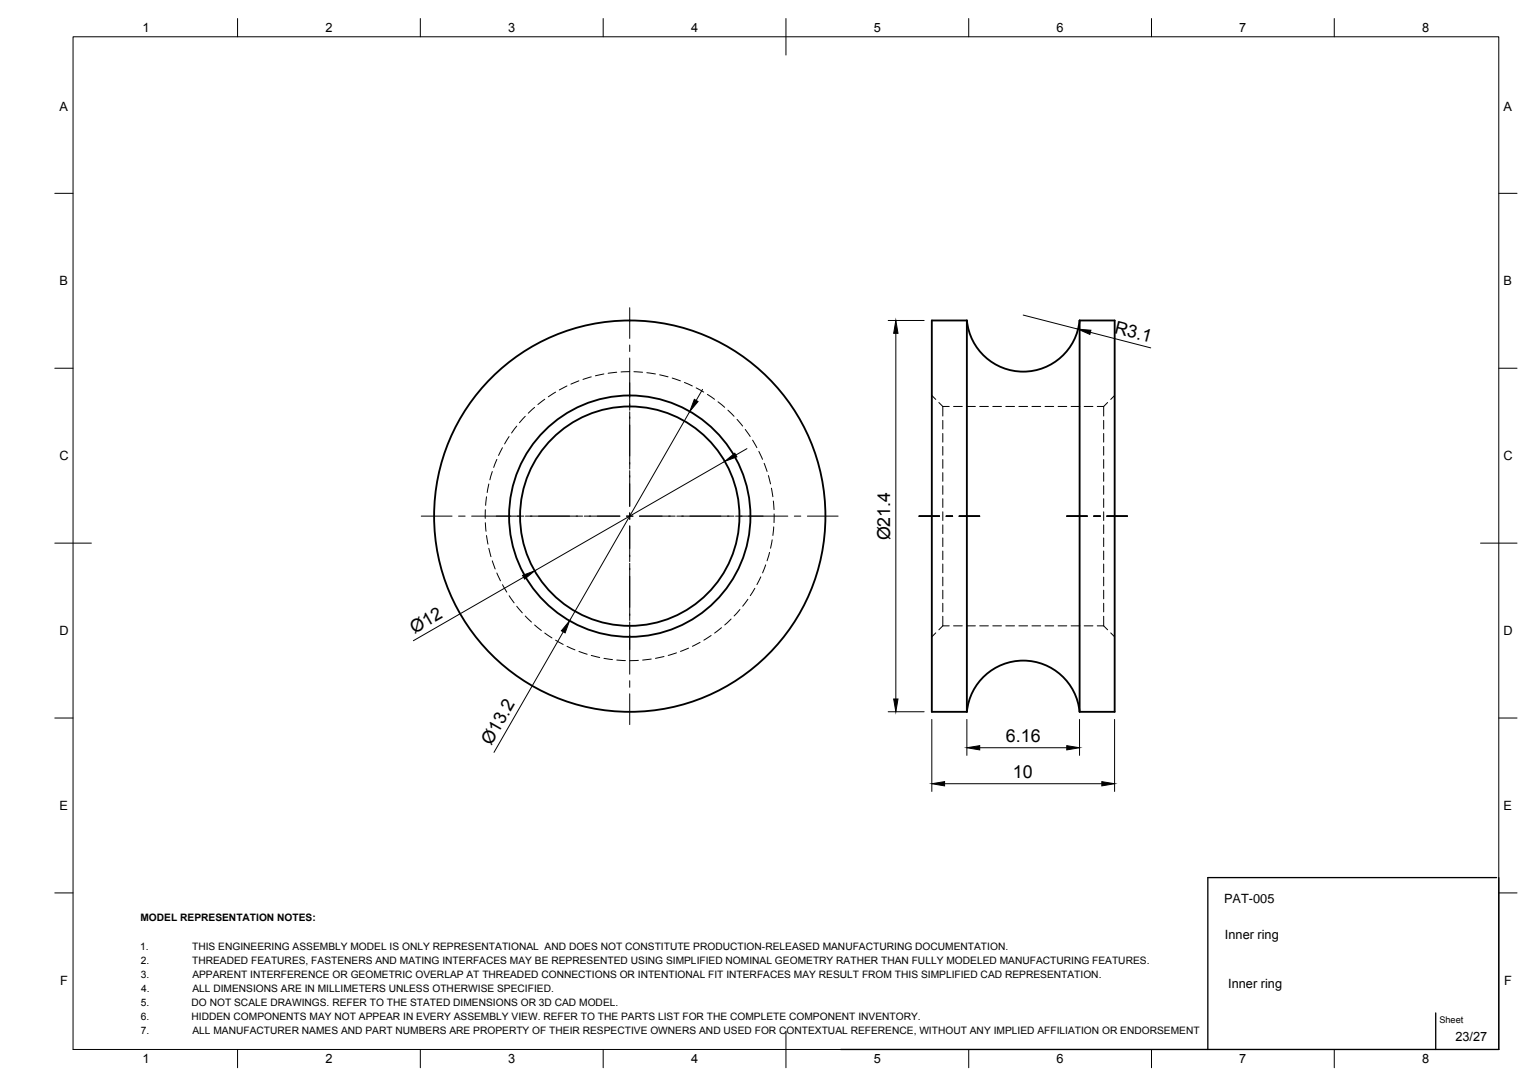
ISO-10303-21;
HEADER;
/* Generated by software containing ST-Developer
 * from STEP Tools, Inc. (www.steptools.com) 
 */

FILE_DESCRIPTION(
/* description */ ('Ball-race swivel caster'),
/* implementation_level */ '2;1');

FILE_NAME(
/* name */ 'Inner ring.step',
/* time_stamp */ '2026-10-29T16:15:51-07:00',
/* author */ (''),
/* organization */ (''),
/* preprocessor_version */ 'ST-DEVELOPER v20.2',
/* originating_system */ 'Autodesk Translation Framework v15.17.0.0',
/* authorisation */ '');

FILE_SCHEMA (('AUTOMOTIVE_DESIGN { 1 0 10303 214 3 1 1 }'));
ENDSEC;

DATA;
#10=MECHANICAL_DESIGN_GEOMETRIC_PRESENTATION_REPRESENTATION('',(#321),#7816);
#30=CONICAL_SURFACE('',#4357,0.63,0.785398163397448);
#31=CONICAL_SURFACE('',#4364,0.63,0.785398163397448);
#190=TOROIDAL_SURFACE('',#4346,1.1,0.309556);
#272=SHAPE_REPRESENTATION_RELATIONSHIP('SRR','None',#7921,#292);
#292=ADVANCED_BREP_SHAPE_REPRESENTATION('',(#356),#7810);
#321=STYLED_ITEM('',(#8097),#356);
#356=MANIFOLD_SOLID_BREP('Body1',#3728);
#427=FACE_BOUND('',#953,.T.);
#428=FACE_BOUND('',#956,.T.);
#506=PLANE('',#4359);
#507=PLANE('',#4362);
#681=FACE_OUTER_BOUND('',#948,.T.);
#682=FACE_OUTER_BOUND('',#949,.T.);
#683=FACE_OUTER_BOUND('',#950,.T.);
#684=FACE_OUTER_BOUND('',#951,.T.);
#685=FACE_OUTER_BOUND('',#952,.T.);
#686=FACE_OUTER_BOUND('',#954,.T.);
#687=FACE_OUTER_BOUND('',#955,.T.);
#688=FACE_OUTER_BOUND('',#957,.T.);
#948=EDGE_LOOP('',(#3217,#3218,#3219,#3220,#3221,#3222));
#949=EDGE_LOOP('',(#3223,#3224,#3225,#3226,#3227));
#950=EDGE_LOOP('',(#3228,#3229,#3230,#3231));
#951=EDGE_LOOP('',(#3232,#3233,#3234,#3235));
#952=EDGE_LOOP('',(#3236));
#953=EDGE_LOOP('',(#3237));
#954=EDGE_LOOP('',(#3238,#3239,#3240,#3241,#3242));
#955=EDGE_LOOP('',(#3243));
#956=EDGE_LOOP('',(#3244));
#957=EDGE_LOOP('',(#3245,#3246,#3247,#3248));
#1148=LINE('',#7228,#1303);
#1149=LINE('',#7234,#1304);
#1150=LINE('',#7238,#1305);
#1151=LINE('',#7244,#1306);
#1152=LINE('',#7249,#1307);
#1303=VECTOR('',#5408,1.070235);
#1304=VECTOR('',#5415,0.6);
#1305=VECTOR('',#5420,0.63);
#1306=VECTOR('',#5429,1.070235);
#1307=VECTOR('',#5436,0.63);
#1512=CIRCLE('',#4347,1.070235);
#1513=CIRCLE('',#4348,1.070235);
#1514=CIRCLE('',#4349,0.309556);
#1515=CIRCLE('',#4350,1.070235);
#1516=CIRCLE('',#4351,1.070235);
#1517=CIRCLE('',#4353,1.070235);
#1518=CIRCLE('',#4355,0.6);
#1519=CIRCLE('',#4356,0.6);
#1520=CIRCLE('',#4358,0.66);
#1521=CIRCLE('',#4361,1.070235);
#1522=CIRCLE('',#4363,0.66);
#1858=VERTEX_POINT('',#7217);
#1859=VERTEX_POINT('',#7218);
#1860=VERTEX_POINT('',#7221);
#1861=VERTEX_POINT('',#7223);
#1862=VERTEX_POINT('',#7227);
#1863=VERTEX_POINT('',#7231);
#1864=VERTEX_POINT('',#7233);
#1865=VERTEX_POINT('',#7237);
#1866=VERTEX_POINT('',#7242);
#1867=VERTEX_POINT('',#7246);
#2328=EDGE_CURVE('',#1858,#1859,#1512,.T.);
#2329=EDGE_CURVE('',#1859,#1858,#1513,.T.);
#2330=EDGE_CURVE('',#1859,#1860,#1514,.T.);
#2331=EDGE_CURVE('',#1861,#1860,#1515,.T.);
#2332=EDGE_CURVE('',#1860,#1861,#1516,.T.);
#2333=EDGE_CURVE('',#1861,#1862,#1148,.T.);
#2334=EDGE_CURVE('',#1862,#1862,#1517,.T.);
#2335=EDGE_CURVE('',#1863,#1863,#1518,.T.);
#2336=EDGE_CURVE('',#1863,#1864,#1149,.T.);
#2337=EDGE_CURVE('',#1864,#1864,#1519,.T.);
#2338=EDGE_CURVE('',#1864,#1865,#1150,.T.);
#2339=EDGE_CURVE('',#1865,#1865,#1520,.T.);
#2340=EDGE_CURVE('',#1866,#1866,#1521,.T.);
#2341=EDGE_CURVE('',#1866,#1858,#1151,.T.);
#2342=EDGE_CURVE('',#1867,#1867,#1522,.T.);
#2343=EDGE_CURVE('',#1867,#1863,#1152,.T.);
#3217=ORIENTED_EDGE('',*,*,#2328,.F.);
#3218=ORIENTED_EDGE('',*,*,#2329,.F.);
#3219=ORIENTED_EDGE('',*,*,#2330,.T.);
#3220=ORIENTED_EDGE('',*,*,#2331,.F.);
#3221=ORIENTED_EDGE('',*,*,#2332,.F.);
#3222=ORIENTED_EDGE('',*,*,#2330,.F.);
#3223=ORIENTED_EDGE('',*,*,#2331,.T.);
#3224=ORIENTED_EDGE('',*,*,#2332,.T.);
#3225=ORIENTED_EDGE('',*,*,#2333,.T.);
#3226=ORIENTED_EDGE('',*,*,#2334,.T.);
#3227=ORIENTED_EDGE('',*,*,#2333,.F.);
#3228=ORIENTED_EDGE('',*,*,#2335,.T.);
#3229=ORIENTED_EDGE('',*,*,#2336,.T.);
#3230=ORIENTED_EDGE('',*,*,#2337,.F.);
#3231=ORIENTED_EDGE('',*,*,#2336,.F.);
#3232=ORIENTED_EDGE('',*,*,#2337,.T.);
#3233=ORIENTED_EDGE('',*,*,#2338,.T.);
#3234=ORIENTED_EDGE('',*,*,#2339,.F.);
#3235=ORIENTED_EDGE('',*,*,#2338,.F.);
#3236=ORIENTED_EDGE('',*,*,#2334,.F.);
#3237=ORIENTED_EDGE('',*,*,#2339,.T.);
#3238=ORIENTED_EDGE('',*,*,#2340,.F.);
#3239=ORIENTED_EDGE('',*,*,#2341,.T.);
#3240=ORIENTED_EDGE('',*,*,#2328,.T.);
#3241=ORIENTED_EDGE('',*,*,#2329,.T.);
#3242=ORIENTED_EDGE('',*,*,#2341,.F.);
#3243=ORIENTED_EDGE('',*,*,#2340,.T.);
#3244=ORIENTED_EDGE('',*,*,#2342,.F.);
#3245=ORIENTED_EDGE('',*,*,#2342,.T.);
#3246=ORIENTED_EDGE('',*,*,#2343,.T.);
#3247=ORIENTED_EDGE('',*,*,#2335,.F.);
#3248=ORIENTED_EDGE('',*,*,#2343,.F.);
#3481=CYLINDRICAL_SURFACE('',#4352,1.070235);
#3482=CYLINDRICAL_SURFACE('',#4354,0.6);
#3483=CYLINDRICAL_SURFACE('',#4360,1.070235);
#3652=ADVANCED_FACE('',(#681),#190,.F.);
#3653=ADVANCED_FACE('',(#682),#3481,.T.);
#3654=ADVANCED_FACE('',(#683),#3482,.F.);
#3655=ADVANCED_FACE('',(#684),#30,.F.);
#3656=ADVANCED_FACE('',(#685,#427),#506,.T.);
#3657=ADVANCED_FACE('',(#686),#3483,.T.);
#3658=ADVANCED_FACE('',(#687,#428),#507,.T.);
#3659=ADVANCED_FACE('',(#688),#31,.F.);
#3728=CLOSED_SHELL('',(#3652,#3653,#3654,#3655,#3656,#3657,#3658,#3659));
#4345=AXIS2_PLACEMENT_3D('',#7215,#5392,#5393);
#4346=AXIS2_PLACEMENT_3D('',#7216,#5394,#5395);
#4347=AXIS2_PLACEMENT_3D('',#7219,#5396,#5397);
#4348=AXIS2_PLACEMENT_3D('',#7220,#5398,#5399);
#4349=AXIS2_PLACEMENT_3D('',#7222,#5400,#5401);
#4350=AXIS2_PLACEMENT_3D('',#7224,#5402,#5403);
#4351=AXIS2_PLACEMENT_3D('',#7225,#5404,#5405);
#4352=AXIS2_PLACEMENT_3D('',#7226,#5406,#5407);
#4353=AXIS2_PLACEMENT_3D('',#7229,#5409,#5410);
#4354=AXIS2_PLACEMENT_3D('',#7230,#5411,#5412);
#4355=AXIS2_PLACEMENT_3D('',#7232,#5413,#5414);
#4356=AXIS2_PLACEMENT_3D('',#7235,#5416,#5417);
#4357=AXIS2_PLACEMENT_3D('',#7236,#5418,#5419);
#4358=AXIS2_PLACEMENT_3D('',#7239,#5421,#5422);
#4359=AXIS2_PLACEMENT_3D('',#7240,#5423,#5424);
#4360=AXIS2_PLACEMENT_3D('',#7241,#5425,#5426);
#4361=AXIS2_PLACEMENT_3D('',#7243,#5427,#5428);
#4362=AXIS2_PLACEMENT_3D('',#7245,#5430,#5431);
#4363=AXIS2_PLACEMENT_3D('',#7247,#5432,#5433);
#4364=AXIS2_PLACEMENT_3D('',#7248,#5434,#5435);
#5392=DIRECTION('axis',(0.,0.,1.));
#5393=DIRECTION('refdir',(1.,0.,0.));
#5394=DIRECTION('center_axis',(0.,-1.,0.));
#5395=DIRECTION('ref_axis',(0.,0.,-1.));
#5396=DIRECTION('center_axis',(0.,-1.,0.));
#5397=DIRECTION('ref_axis',(1.,0.,0.));
#5398=DIRECTION('center_axis',(0.,-1.,0.));
#5399=DIRECTION('ref_axis',(1.,0.,0.));
#5400=DIRECTION('center_axis',(1.,0.,1.22464679914735E-16));
#5401=DIRECTION('ref_axis',(-1.22464679914735E-16,0.,1.));
#5402=DIRECTION('center_axis',(0.,1.,0.));
#5403=DIRECTION('ref_axis',(1.,0.,0.));
#5404=DIRECTION('center_axis',(0.,1.,0.));
#5405=DIRECTION('ref_axis',(1.,0.,0.));
#5406=DIRECTION('center_axis',(0.,-1.,0.));
#5407=DIRECTION('ref_axis',(1.,0.,0.));
#5408=DIRECTION('',(0.,1.,0.));
#5409=DIRECTION('center_axis',(0.,-1.,0.));
#5410=DIRECTION('ref_axis',(1.,0.,0.));
#5411=DIRECTION('center_axis',(0.,-1.,0.));
#5412=DIRECTION('ref_axis',(1.,0.,0.));
#5413=DIRECTION('center_axis',(0.,-1.,0.));
#5414=DIRECTION('ref_axis',(1.,0.,0.));
#5415=DIRECTION('',(0.,1.,0.));
#5416=DIRECTION('center_axis',(0.,-1.,0.));
#5417=DIRECTION('ref_axis',(1.,0.,0.));
#5418=DIRECTION('center_axis',(0.,1.,0.));
#5419=DIRECTION('ref_axis',(1.,0.,0.));
#5420=DIRECTION('',(-0.707106781186548,0.707106781186547,-8.65956056235493E-17));
#5421=DIRECTION('center_axis',(0.,-1.,0.));
#5422=DIRECTION('ref_axis',(1.,0.,0.));
#5423=DIRECTION('center_axis',(0.,1.,0.));
#5424=DIRECTION('ref_axis',(0.,0.,1.));
#5425=DIRECTION('center_axis',(0.,-1.,0.));
#5426=DIRECTION('ref_axis',(1.,0.,0.));
#5427=DIRECTION('center_axis',(0.,-1.,0.));
#5428=DIRECTION('ref_axis',(1.,0.,0.));
#5429=DIRECTION('',(0.,1.,0.));
#5430=DIRECTION('center_axis',(0.,-1.,0.));
#5431=DIRECTION('ref_axis',(0.,0.,-1.));
#5432=DIRECTION('center_axis',(0.,-1.,0.));
#5433=DIRECTION('ref_axis',(1.,0.,0.));
#5434=DIRECTION('center_axis',(0.,-1.,0.));
#5435=DIRECTION('ref_axis',(1.,0.,0.));
#5436=DIRECTION('',(0.707106781186548,0.707106781186547,8.65956056235493E-17));
#7215=CARTESIAN_POINT('',(0.,0.,0.));
#7216=CARTESIAN_POINT('Origin',(0.,0.,0.));
#7217=CARTESIAN_POINT('',(-1.070235,-0.308121667383195,-1.31065986708547E-16));
#7218=CARTESIAN_POINT('',(-1.31065986708547E-16,-0.308121667383195,1.070235));
#7219=CARTESIAN_POINT('Origin',(0.,-0.308121667383195,0.));
#7220=CARTESIAN_POINT('Origin',(0.,-0.308121667383195,0.));
#7221=CARTESIAN_POINT('',(-1.31065986708547E-16,0.308121667383195,1.070235));
#7222=CARTESIAN_POINT('Origin',(-1.34711147906209E-16,0.,1.1));
#7223=CARTESIAN_POINT('',(-1.070235,0.308121667383195,1.31065986708547E-16));
#7224=CARTESIAN_POINT('Origin',(0.,0.308121667383195,0.));
#7225=CARTESIAN_POINT('Origin',(0.,0.308121667383195,0.));
#7226=CARTESIAN_POINT('Origin',(0.,0.,0.));
#7227=CARTESIAN_POINT('',(-1.070235,0.5,-1.31065986708547E-16));
#7228=CARTESIAN_POINT('',(-1.070235,0.,-1.31065986708547E-16));
#7229=CARTESIAN_POINT('Origin',(0.,0.5,0.));
#7230=CARTESIAN_POINT('Origin',(0.,0.,0.));
#7231=CARTESIAN_POINT('',(-0.6,-0.44,-7.34788079488412E-17));
#7232=CARTESIAN_POINT('Origin',(0.,-0.44,0.));
#7233=CARTESIAN_POINT('',(-0.6,0.44,-7.34788079488412E-17));
#7234=CARTESIAN_POINT('',(-0.6,0.,-7.34788079488412E-17));
#7235=CARTESIAN_POINT('Origin',(0.,0.44,0.));
#7236=CARTESIAN_POINT('Origin',(0.,0.47,0.));
#7237=CARTESIAN_POINT('',(-0.66,0.5,-8.08266887437253E-17));
#7238=CARTESIAN_POINT('',(-0.63,0.47,-7.71527483462832E-17));
#7239=CARTESIAN_POINT('Origin',(0.,0.5,0.));
#7240=CARTESIAN_POINT('Origin',(1.070235,0.5,0.));
#7241=CARTESIAN_POINT('Origin',(0.,0.,0.));
#7242=CARTESIAN_POINT('',(-1.070235,-0.5,-1.31065986708547E-16));
#7243=CARTESIAN_POINT('Origin',(0.,-0.5,0.));
#7244=CARTESIAN_POINT('',(-1.070235,0.,-1.31065986708547E-16));
#7245=CARTESIAN_POINT('Origin',(0.66,-0.5,0.));
#7246=CARTESIAN_POINT('',(-0.66,-0.5,-8.08266887437253E-17));
#7247=CARTESIAN_POINT('Origin',(0.,-0.5,0.));
#7248=CARTESIAN_POINT('Origin',(0.,-0.47,0.));
#7249=CARTESIAN_POINT('',(-0.63,-0.47,-7.71527483462832E-17));
#7783=UNCERTAINTY_MEASURE_WITH_UNIT(LENGTH_MEASURE(0.001),#7817,
'DISTANCE_ACCURACY_VALUE',
'Maximum model space distance between geometric entities at asserted c
onnectivities');
#7789=UNCERTAINTY_MEASURE_WITH_UNIT(LENGTH_MEASURE(0.001),#7817,
'DISTANCE_ACCURACY_VALUE',
'Maximum model space distance between geometric entities at asserted c
onnectivities');
#7810=(
GEOMETRIC_REPRESENTATION_CONTEXT(3)
GLOBAL_UNCERTAINTY_ASSIGNED_CONTEXT((#7783))
GLOBAL_UNIT_ASSIGNED_CONTEXT((#7817,#7819,#7820))
REPRESENTATION_CONTEXT('','3D')
);
#7816=(
GEOMETRIC_REPRESENTATION_CONTEXT(3)
GLOBAL_UNCERTAINTY_ASSIGNED_CONTEXT((#7789))
GLOBAL_UNIT_ASSIGNED_CONTEXT((#7817,#7819,#7820))
REPRESENTATION_CONTEXT('','3D')
);
#7817=(
LENGTH_UNIT()
NAMED_UNIT(*)
SI_UNIT(.CENTI.,.METRE.)
);
#7819=(
NAMED_UNIT(*)
PLANE_ANGLE_UNIT()
SI_UNIT($,.RADIAN.)
);
#7820=(
NAMED_UNIT(*)
SI_UNIT($,.STERADIAN.)
SOLID_ANGLE_UNIT()
);
#7841=SHAPE_DEFINITION_REPRESENTATION(#7882,#7921);
#7882=PRODUCT_DEFINITION_SHAPE('',$,#7948);
#7921=SHAPE_REPRESENTATION('',(#4345),#7810);
#7927=PRODUCT_DEFINITION_CONTEXT('part definition',#8007,'design');
#7948=PRODUCT_DEFINITION('Inner ring','Inner ring',#7974,#7927);
#7974=PRODUCT_DEFINITION_FORMATION('',$,#8029);
#8007=APPLICATION_CONTEXT(
'Core Data for Automotive Mechanical Design Process');
#8008=PRODUCT_CONTEXT('part definition',#8007,'mechanical');
#8029=PRODUCT('Inner ring','Inner ring','Inner ring',(#8008));
#8091=COLOUR_RGB('Grey',0.48,0.52,0.57);
#8092=FILL_AREA_STYLE_COLOUR('',#8091);
#8093=FILL_AREA_STYLE('',(#8092));
#8094=SURFACE_STYLE_FILL_AREA(#8093);
#8095=SURFACE_SIDE_STYLE('',(#8094));
#8096=SURFACE_STYLE_USAGE(.BOTH.,#8095);
#8097=PRESENTATION_STYLE_ASSIGNMENT((#8096));
ENDSEC;
END-ISO-10303-21;
